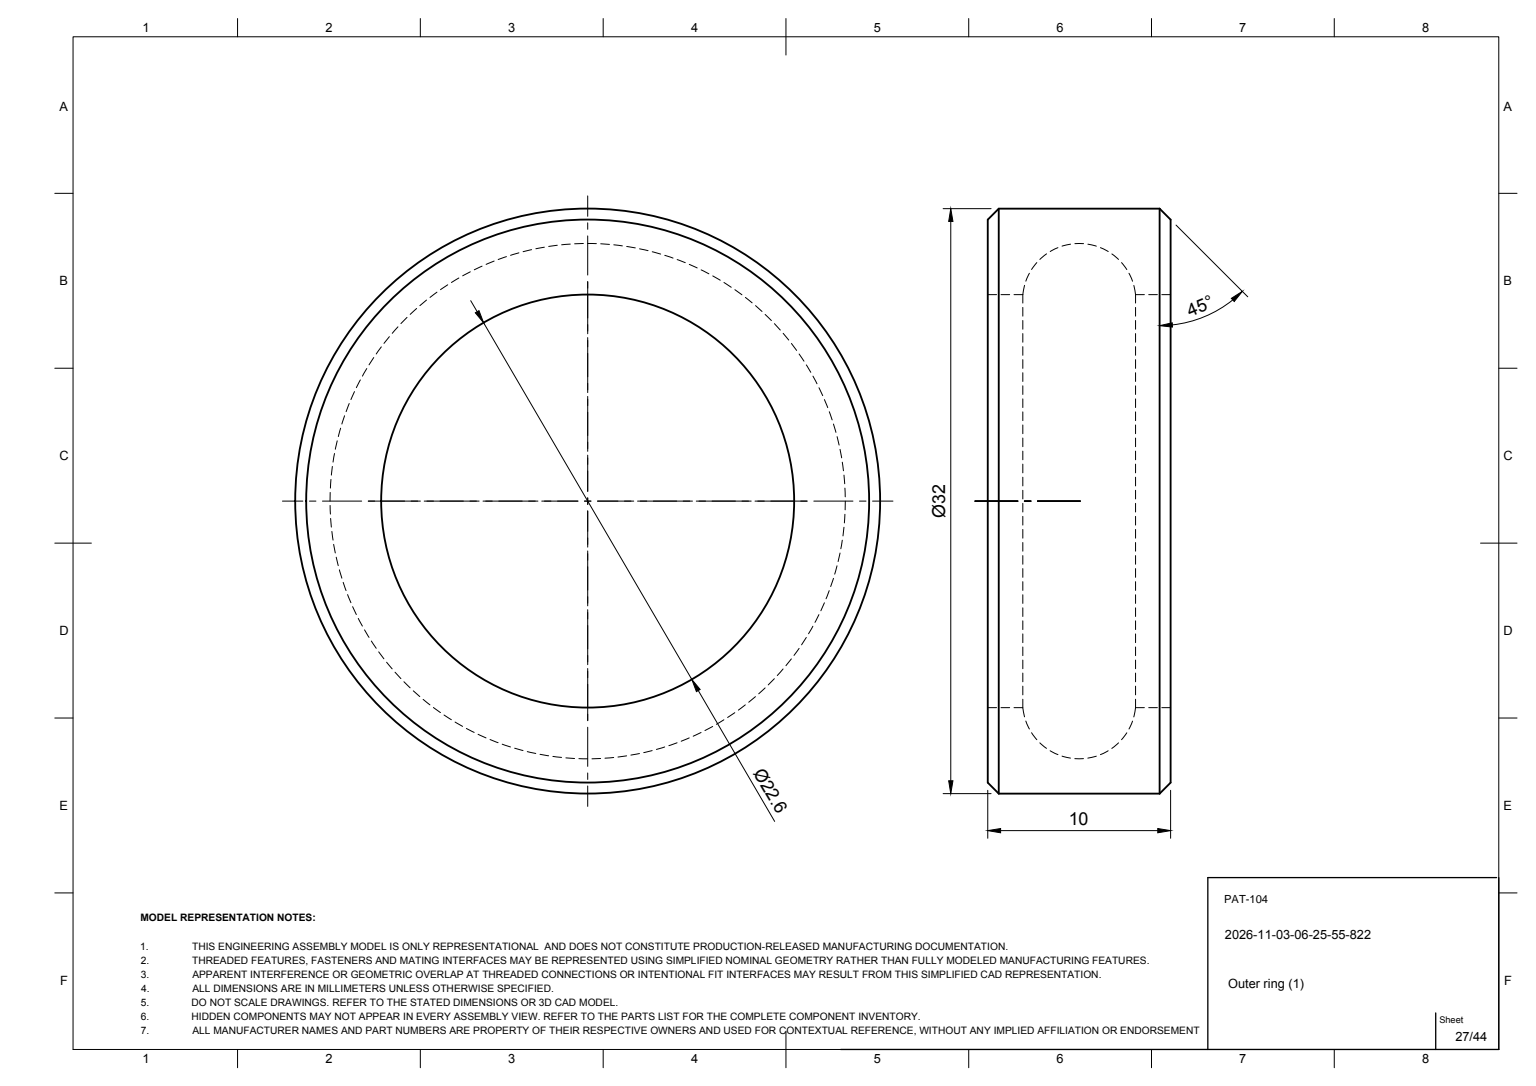
ISO-10303-21;
HEADER;
/* Generated by software containing ST-Developer
 * from STEP Tools, Inc. (www.steptools.com) 
 */

FILE_DESCRIPTION(
/* description */ ('Timing belt drive module 2 mm Pitch Timing 20T-40T'),

/* implementation_level */ '2;1');

FILE_NAME(
/* name */ 'Outer ring (1).step',
/* time_stamp */ '2026-10-28T03:25:12-07:00',
/* author */ (''),
/* organization */ (''),
/* preprocessor_version */ 'ST-DEVELOPER v20.2',
/* originating_system */ 'Autodesk Translation Framework v15.17.0.0',
/* authorisation */ '');

FILE_SCHEMA (('AUTOMOTIVE_DESIGN { 1 0 10303 214 3 1 1 }'));
ENDSEC;

DATA;
#10=MECHANICAL_DESIGN_GEOMETRIC_PRESENTATION_REPRESENTATION('',(#555),#17830);
#425=CONICAL_SURFACE('',#10073,1.57,0.785398163397449);
#426=CONICAL_SURFACE('',#10077,1.57,0.785398163397449);
#437=TOROIDAL_SURFACE('',#10062,1.1,0.309556);
#461=SHAPE_REPRESENTATION_RELATIONSHIP('SRR','None',#18033,#504);
#504=ADVANCED_BREP_SHAPE_REPRESENTATION('',(#612),#17808);
#555=STYLED_ITEM('',(#18317),#612);
#612=MANIFOLD_SOLID_BREP('Body1',#9013);
#722=FACE_BOUND('',#1815,.T.);
#723=FACE_BOUND('',#1820,.T.);
#884=PLANE('',#10070);
#885=PLANE('',#10079);
#1206=FACE_OUTER_BOUND('',#1812,.T.);
#1207=FACE_OUTER_BOUND('',#1813,.T.);
#1208=FACE_OUTER_BOUND('',#1814,.T.);
#1209=FACE_OUTER_BOUND('',#1816,.T.);
#1210=FACE_OUTER_BOUND('',#1817,.T.);
#1211=FACE_OUTER_BOUND('',#1818,.T.);
#1212=FACE_OUTER_BOUND('',#1819,.T.);
#1213=FACE_OUTER_BOUND('',#1821,.T.);
#1812=EDGE_LOOP('',(#6855,#6856,#6857,#6858,#6859,#6860));
#1813=EDGE_LOOP('',(#6861,#6862,#6863,#6864,#6865));
#1814=EDGE_LOOP('',(#6866));
#1815=EDGE_LOOP('',(#6867));
#1816=EDGE_LOOP('',(#6868,#6869,#6870,#6871));
#1817=EDGE_LOOP('',(#6872,#6873,#6874,#6875));
#1818=EDGE_LOOP('',(#6876,#6877,#6878,#6879));
#1819=EDGE_LOOP('',(#6880));
#1820=EDGE_LOOP('',(#6881));
#1821=EDGE_LOOP('',(#6882,#6883,#6884,#6885,#6886));
#2409=CIRCLE('',#10063,1.129765);
#2410=CIRCLE('',#10064,1.129765);
#2411=CIRCLE('',#10065,0.309556);
#2412=CIRCLE('',#10066,1.129765);
#2413=CIRCLE('',#10067,1.129765);
#2414=CIRCLE('',#10069,1.129765);
#2415=CIRCLE('',#10071,1.54);
#2416=CIRCLE('',#10072,1.129765);
#2417=CIRCLE('',#10074,1.6);
#2418=CIRCLE('',#10076,1.6);
#2419=CIRCLE('',#10078,1.54);
#3044=LINE('',#15410,#3522);
#3045=LINE('',#15419,#3523);
#3046=LINE('',#15423,#3524);
#3047=LINE('',#15427,#3525);
#3048=LINE('',#15430,#3526);
#3522=VECTOR('',#12171,1.129765);
#3523=VECTOR('',#12182,1.57);
#3524=VECTOR('',#12187,1.6);
#3525=VECTOR('',#12192,1.57);
#3526=VECTOR('',#12197,1.129765);
#4114=VERTEX_POINT('',#15398);
#4115=VERTEX_POINT('',#15399);
#4116=VERTEX_POINT('',#15402);
#4117=VERTEX_POINT('',#15404);
#4118=VERTEX_POINT('',#15408);
#4119=VERTEX_POINT('',#15412);
#4120=VERTEX_POINT('',#15414);
#4121=VERTEX_POINT('',#15417);
#4122=VERTEX_POINT('',#15421);
#4123=VERTEX_POINT('',#15425);
#5110=EDGE_CURVE('',#4114,#4115,#2409,.T.);
#5111=EDGE_CURVE('',#4115,#4114,#2410,.T.);
#5112=EDGE_CURVE('',#4115,#4116,#2411,.T.);
#5113=EDGE_CURVE('',#4117,#4116,#2412,.T.);
#5114=EDGE_CURVE('',#4116,#4117,#2413,.T.);
#5115=EDGE_CURVE('',#4118,#4118,#2414,.T.);
#5116=EDGE_CURVE('',#4118,#4117,#3044,.T.);
#5117=EDGE_CURVE('',#4119,#4119,#2415,.T.);
#5118=EDGE_CURVE('',#4120,#4120,#2416,.T.);
#5119=EDGE_CURVE('',#4121,#4121,#2417,.T.);
#5120=EDGE_CURVE('',#4121,#4119,#3045,.T.);
#5121=EDGE_CURVE('',#4122,#4122,#2418,.T.);
#5122=EDGE_CURVE('',#4122,#4121,#3046,.T.);
#5123=EDGE_CURVE('',#4123,#4123,#2419,.T.);
#5124=EDGE_CURVE('',#4123,#4122,#3047,.T.);
#5125=EDGE_CURVE('',#4114,#4120,#3048,.T.);
#6855=ORIENTED_EDGE('',*,*,#5110,.F.);
#6856=ORIENTED_EDGE('',*,*,#5111,.F.);
#6857=ORIENTED_EDGE('',*,*,#5112,.T.);
#6858=ORIENTED_EDGE('',*,*,#5113,.F.);
#6859=ORIENTED_EDGE('',*,*,#5114,.F.);
#6860=ORIENTED_EDGE('',*,*,#5112,.F.);
#6861=ORIENTED_EDGE('',*,*,#5115,.T.);
#6862=ORIENTED_EDGE('',*,*,#5116,.T.);
#6863=ORIENTED_EDGE('',*,*,#5113,.T.);
#6864=ORIENTED_EDGE('',*,*,#5114,.T.);
#6865=ORIENTED_EDGE('',*,*,#5116,.F.);
#6866=ORIENTED_EDGE('',*,*,#5117,.F.);
#6867=ORIENTED_EDGE('',*,*,#5118,.T.);
#6868=ORIENTED_EDGE('',*,*,#5119,.F.);
#6869=ORIENTED_EDGE('',*,*,#5120,.T.);
#6870=ORIENTED_EDGE('',*,*,#5117,.T.);
#6871=ORIENTED_EDGE('',*,*,#5120,.F.);
#6872=ORIENTED_EDGE('',*,*,#5121,.F.);
#6873=ORIENTED_EDGE('',*,*,#5122,.T.);
#6874=ORIENTED_EDGE('',*,*,#5119,.T.);
#6875=ORIENTED_EDGE('',*,*,#5122,.F.);
#6876=ORIENTED_EDGE('',*,*,#5123,.F.);
#6877=ORIENTED_EDGE('',*,*,#5124,.T.);
#6878=ORIENTED_EDGE('',*,*,#5121,.T.);
#6879=ORIENTED_EDGE('',*,*,#5124,.F.);
#6880=ORIENTED_EDGE('',*,*,#5123,.T.);
#6881=ORIENTED_EDGE('',*,*,#5115,.F.);
#6882=ORIENTED_EDGE('',*,*,#5110,.T.);
#6883=ORIENTED_EDGE('',*,*,#5111,.T.);
#6884=ORIENTED_EDGE('',*,*,#5125,.T.);
#6885=ORIENTED_EDGE('',*,*,#5118,.F.);
#6886=ORIENTED_EDGE('',*,*,#5125,.F.);
#8285=CYLINDRICAL_SURFACE('',#10068,1.129765);
#8286=CYLINDRICAL_SURFACE('',#10075,1.6);
#8287=CYLINDRICAL_SURFACE('',#10080,1.129765);
#8704=ADVANCED_FACE('',(#1206),#437,.F.);
#8705=ADVANCED_FACE('',(#1207),#8285,.F.);
#8706=ADVANCED_FACE('',(#1208,#722),#884,.T.);
#8707=ADVANCED_FACE('',(#1209),#425,.T.);
#8708=ADVANCED_FACE('',(#1210),#8286,.T.);
#8709=ADVANCED_FACE('',(#1211),#426,.T.);
#8710=ADVANCED_FACE('',(#1212,#723),#885,.T.);
#8711=ADVANCED_FACE('',(#1213),#8287,.F.);
#9013=CLOSED_SHELL('',(#8704,#8705,#8706,#8707,#8708,#8709,#8710,#8711));
#10061=AXIS2_PLACEMENT_3D('',#15396,#12153,#12154);
#10062=AXIS2_PLACEMENT_3D('',#15397,#12155,#12156);
#10063=AXIS2_PLACEMENT_3D('',#15400,#12157,#12158);
#10064=AXIS2_PLACEMENT_3D('',#15401,#12159,#12160);
#10065=AXIS2_PLACEMENT_3D('',#15403,#12161,#12162);
#10066=AXIS2_PLACEMENT_3D('',#15405,#12163,#12164);
#10067=AXIS2_PLACEMENT_3D('',#15406,#12165,#12166);
#10068=AXIS2_PLACEMENT_3D('',#15407,#12167,#12168);
#10069=AXIS2_PLACEMENT_3D('',#15409,#12169,#12170);
#10070=AXIS2_PLACEMENT_3D('',#15411,#12172,#12173);
#10071=AXIS2_PLACEMENT_3D('',#15413,#12174,#12175);
#10072=AXIS2_PLACEMENT_3D('',#15415,#12176,#12177);
#10073=AXIS2_PLACEMENT_3D('',#15416,#12178,#12179);
#10074=AXIS2_PLACEMENT_3D('',#15418,#12180,#12181);
#10075=AXIS2_PLACEMENT_3D('',#15420,#12183,#12184);
#10076=AXIS2_PLACEMENT_3D('',#15422,#12185,#12186);
#10077=AXIS2_PLACEMENT_3D('',#15424,#12188,#12189);
#10078=AXIS2_PLACEMENT_3D('',#15426,#12190,#12191);
#10079=AXIS2_PLACEMENT_3D('',#15428,#12193,#12194);
#10080=AXIS2_PLACEMENT_3D('',#15429,#12195,#12196);
#12153=DIRECTION('axis',(0.,0.,1.));
#12154=DIRECTION('refdir',(1.,0.,0.));
#12155=DIRECTION('center_axis',(0.,-1.,0.));
#12156=DIRECTION('ref_axis',(0.,0.,-1.));
#12157=DIRECTION('center_axis',(0.,-1.,0.));
#12158=DIRECTION('ref_axis',(1.,0.,0.));
#12159=DIRECTION('center_axis',(0.,-1.,0.));
#12160=DIRECTION('ref_axis',(1.,0.,0.));
#12161=DIRECTION('center_axis',(1.,0.,1.22464679914735E-16));
#12162=DIRECTION('ref_axis',(-1.22464679914735E-16,0.,1.));
#12163=DIRECTION('center_axis',(0.,1.,0.));
#12164=DIRECTION('ref_axis',(1.,0.,0.));
#12165=DIRECTION('center_axis',(0.,1.,0.));
#12166=DIRECTION('ref_axis',(1.,0.,0.));
#12167=DIRECTION('center_axis',(0.,-1.,0.));
#12168=DIRECTION('ref_axis',(1.,0.,0.));
#12169=DIRECTION('center_axis',(0.,-1.,0.));
#12170=DIRECTION('ref_axis',(1.,0.,0.));
#12171=DIRECTION('',(0.,1.,0.));
#12172=DIRECTION('center_axis',(0.,1.,0.));
#12173=DIRECTION('ref_axis',(0.,0.,1.));
#12174=DIRECTION('center_axis',(0.,-1.,0.));
#12175=DIRECTION('ref_axis',(1.,0.,0.));
#12176=DIRECTION('center_axis',(0.,-1.,0.));
#12177=DIRECTION('ref_axis',(1.,0.,0.));
#12178=DIRECTION('center_axis',(0.,-1.,0.));
#12179=DIRECTION('ref_axis',(1.,0.,0.));
#12180=DIRECTION('center_axis',(0.,-1.,0.));
#12181=DIRECTION('ref_axis',(1.,0.,0.));
#12182=DIRECTION('',(0.707106781186548,0.707106781186547,8.65956056235494E-17));
#12183=DIRECTION('center_axis',(0.,-1.,0.));
#12184=DIRECTION('ref_axis',(1.,0.,0.));
#12185=DIRECTION('center_axis',(0.,-1.,0.));
#12186=DIRECTION('ref_axis',(1.,0.,0.));
#12187=DIRECTION('',(0.,1.,0.));
#12188=DIRECTION('center_axis',(0.,1.,0.));
#12189=DIRECTION('ref_axis',(1.,0.,0.));
#12190=DIRECTION('center_axis',(0.,-1.,0.));
#12191=DIRECTION('ref_axis',(1.,0.,0.));
#12192=DIRECTION('',(-0.707106781186548,0.707106781186547,-8.65956056235494E-17));
#12193=DIRECTION('center_axis',(0.,-1.,0.));
#12194=DIRECTION('ref_axis',(0.,0.,-1.));
#12195=DIRECTION('center_axis',(0.,-1.,0.));
#12196=DIRECTION('ref_axis',(1.,0.,0.));
#12197=DIRECTION('',(0.,1.,0.));
#15396=CARTESIAN_POINT('',(0.,0.,0.));
#15397=CARTESIAN_POINT('Origin',(0.,0.,0.));
#15398=CARTESIAN_POINT('',(-1.129765,0.308121667383195,-1.38356309103871E-16));
#15399=CARTESIAN_POINT('',(-1.38356309103871E-16,0.308121667383195,1.129765));
#15400=CARTESIAN_POINT('Origin',(0.,0.308121667383195,0.));
#15401=CARTESIAN_POINT('Origin',(0.,0.308121667383195,0.));
#15402=CARTESIAN_POINT('',(-1.38356309103871E-16,-0.308121667383195,1.129765));
#15403=CARTESIAN_POINT('Origin',(-1.34711147906209E-16,0.,1.1));
#15404=CARTESIAN_POINT('',(-1.129765,-0.308121667383195,1.38356309103871E-16));
#15405=CARTESIAN_POINT('Origin',(0.,-0.308121667383195,0.));
#15406=CARTESIAN_POINT('Origin',(0.,-0.308121667383195,0.));
#15407=CARTESIAN_POINT('Origin',(0.,0.,0.));
#15408=CARTESIAN_POINT('',(-1.129765,-0.5,-1.38356309103871E-16));
#15409=CARTESIAN_POINT('Origin',(0.,-0.5,0.));
#15410=CARTESIAN_POINT('',(-1.129765,0.,-1.38356309103871E-16));
#15411=CARTESIAN_POINT('Origin',(1.54,0.5,0.));
#15412=CARTESIAN_POINT('',(-1.54,0.5,-1.88595607068692E-16));
#15413=CARTESIAN_POINT('Origin',(0.,0.5,0.));
#15414=CARTESIAN_POINT('',(-1.129765,0.5,-1.38356309103871E-16));
#15415=CARTESIAN_POINT('Origin',(0.,0.5,0.));
#15416=CARTESIAN_POINT('Origin',(0.,0.47,0.));
#15417=CARTESIAN_POINT('',(-1.6,0.44,-1.95943487863577E-16));
#15418=CARTESIAN_POINT('Origin',(0.,0.44,0.));
#15419=CARTESIAN_POINT('',(-1.57,0.47,-1.92269547466134E-16));
#15420=CARTESIAN_POINT('Origin',(0.,0.,0.));
#15421=CARTESIAN_POINT('',(-1.6,-0.44,-1.95943487863577E-16));
#15422=CARTESIAN_POINT('Origin',(0.,-0.44,0.));
#15423=CARTESIAN_POINT('',(-1.6,0.,-1.95943487863577E-16));
#15424=CARTESIAN_POINT('Origin',(0.,-0.47,0.));
#15425=CARTESIAN_POINT('',(-1.54,-0.5,-1.88595607068692E-16));
#15426=CARTESIAN_POINT('Origin',(0.,-0.5,0.));
#15427=CARTESIAN_POINT('',(-1.57,-0.47,-1.92269547466134E-16));
#15428=CARTESIAN_POINT('Origin',(1.129765,-0.5,0.));
#15429=CARTESIAN_POINT('Origin',(0.,0.,0.));
#15430=CARTESIAN_POINT('',(-1.129765,0.,-1.38356309103871E-16));
#17758=UNCERTAINTY_MEASURE_WITH_UNIT(LENGTH_MEASURE(0.001),#17831,
'DISTANCE_ACCURACY_VALUE',
'Maximum model space distance between geometric entities at asserted c
onnectivities');
#17780=UNCERTAINTY_MEASURE_WITH_UNIT(LENGTH_MEASURE(0.001),#17831,
'DISTANCE_ACCURACY_VALUE',
'Maximum model space distance between geometric entities at asserted c
onnectivities');
#17808=(
GEOMETRIC_REPRESENTATION_CONTEXT(3)
GLOBAL_UNCERTAINTY_ASSIGNED_CONTEXT((#17758))
GLOBAL_UNIT_ASSIGNED_CONTEXT((#17831,#17833,#17834))
REPRESENTATION_CONTEXT('','3D')
);
#17830=(
GEOMETRIC_REPRESENTATION_CONTEXT(3)
GLOBAL_UNCERTAINTY_ASSIGNED_CONTEXT((#17780))
GLOBAL_UNIT_ASSIGNED_CONTEXT((#17831,#17833,#17834))
REPRESENTATION_CONTEXT('','3D')
);
#17831=(
LENGTH_UNIT()
NAMED_UNIT(*)
SI_UNIT(.CENTI.,.METRE.)
);
#17833=(
NAMED_UNIT(*)
PLANE_ANGLE_UNIT()
SI_UNIT($,.RADIAN.)
);
#17834=(
NAMED_UNIT(*)
SI_UNIT($,.STERADIAN.)
SOLID_ANGLE_UNIT()
);
#17862=SHAPE_DEFINITION_REPRESENTATION(#17916,#18033);
#17916=PRODUCT_DEFINITION_SHAPE('',$,#18083);
#18033=SHAPE_REPRESENTATION('',(#10061),#17808);
#18055=PRODUCT_DEFINITION_CONTEXT('part definition',#18204,'design');
#18083=PRODUCT_DEFINITION('Outer ring (1)','Outer ring (1)',#18132,#18055);
#18132=PRODUCT_DEFINITION_FORMATION('',$,#18233);
#18204=APPLICATION_CONTEXT(
'Core Data for Automotive Mechanical Design Process');
#18205=PRODUCT_CONTEXT('part definition',#18204,'mechanical');
#18233=PRODUCT('Outer ring (1)','Outer ring (1)','Outer ring (1)',(#18205));
#18311=COLOUR_RGB('Grey',0.48,0.52,0.57);
#18312=FILL_AREA_STYLE_COLOUR('',#18311);
#18313=FILL_AREA_STYLE('',(#18312));
#18314=SURFACE_STYLE_FILL_AREA(#18313);
#18315=SURFACE_SIDE_STYLE('',(#18314));
#18316=SURFACE_STYLE_USAGE(.BOTH.,#18315);
#18317=PRESENTATION_STYLE_ASSIGNMENT((#18316));
ENDSEC;
END-ISO-10303-21;
